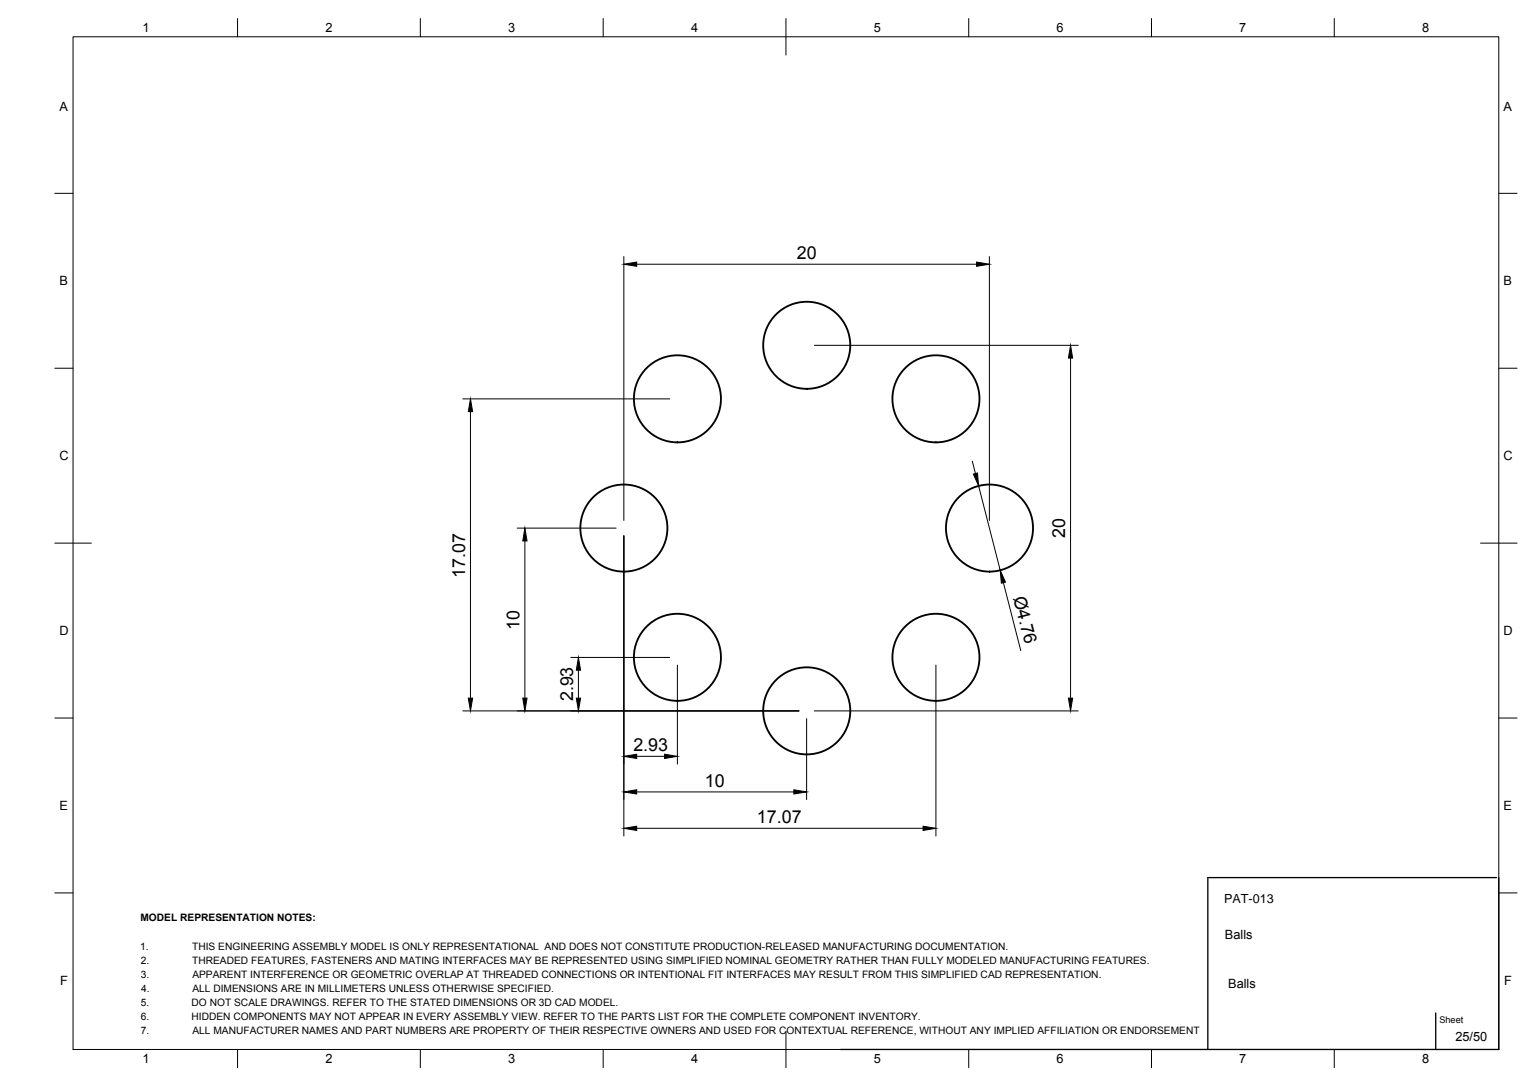
ISO-10303-21;
HEADER;
/* Generated by software containing ST-Developer
 * from STEP Tools, Inc. (www.steptools.com) 
 */

FILE_DESCRIPTION(
/* description */ ('Belt-driven linear axis on 2020 extrusion'),
/* implementation_level */ '2;1');

FILE_NAME(
/* name */ 'Balls.step',
/* time_stamp */ '2026-10-28T03:26:09-07:00',
/* author */ (''),
/* organization */ (''),
/* preprocessor_version */ 'ST-DEVELOPER v20.2',
/* originating_system */ 'Autodesk Translation Framework v15.17.0.0',
/* authorisation */ '');

FILE_SCHEMA (('AUTOMOTIVE_DESIGN { 1 0 10303 214 3 1 1 }'));
ENDSEC;

DATA;
#10=MECHANICAL_DESIGN_GEOMETRIC_PRESENTATION_REPRESENTATION('',(#628,#629,#630,#631,#632,#633,#634,#635),#20096);
#481=SPHERICAL_SURFACE('',#11958,0.23815);
#482=SPHERICAL_SURFACE('',#11960,0.23815);
#483=SPHERICAL_SURFACE('',#11962,0.23815);
#484=SPHERICAL_SURFACE('',#11964,0.23815);
#485=SPHERICAL_SURFACE('',#11966,0.23815);
#486=SPHERICAL_SURFACE('',#11968,0.23815);
#487=SPHERICAL_SURFACE('',#11970,0.23815);
#488=SPHERICAL_SURFACE('',#11972,0.23815);
#534=SHAPE_REPRESENTATION_RELATIONSHIP('SRR','None',#20331,#580);
#580=ADVANCED_BREP_SHAPE_REPRESENTATION('',(#684,#685,#686,#687,#688,#689,
#690,#691),#20062);
#628=STYLED_ITEM('',(#20650),#684);
#629=STYLED_ITEM('',(#20650),#685);
#630=STYLED_ITEM('',(#20650),#686);
#631=STYLED_ITEM('',(#20650),#687);
#632=STYLED_ITEM('',(#20650),#688);
#633=STYLED_ITEM('',(#20650),#689);
#634=STYLED_ITEM('',(#20650),#690);
#635=STYLED_ITEM('',(#20650),#691);
#684=MANIFOLD_SOLID_BREP('Body1',#10941);
#685=MANIFOLD_SOLID_BREP('Body2',#10942);
#686=MANIFOLD_SOLID_BREP('Body3',#10943);
#687=MANIFOLD_SOLID_BREP('Body4',#10944);
#688=MANIFOLD_SOLID_BREP('Body5',#10945);
#689=MANIFOLD_SOLID_BREP('Body6',#10946);
#690=MANIFOLD_SOLID_BREP('Body7',#10947);
#691=MANIFOLD_SOLID_BREP('Body8',#10948);
#1480=FACE_OUTER_BOUND('',#2192,.T.);
#1481=FACE_OUTER_BOUND('',#2193,.T.);
#1482=FACE_OUTER_BOUND('',#2194,.T.);
#1483=FACE_OUTER_BOUND('',#2195,.T.);
#1484=FACE_OUTER_BOUND('',#2196,.T.);
#1485=FACE_OUTER_BOUND('',#2197,.T.);
#1486=FACE_OUTER_BOUND('',#2198,.T.);
#1487=FACE_OUTER_BOUND('',#2199,.T.);
#2192=EDGE_LOOP('',(#8289,#8290));
#2193=EDGE_LOOP('',(#8291,#8292));
#2194=EDGE_LOOP('',(#8293,#8294));
#2195=EDGE_LOOP('',(#8295,#8296));
#2196=EDGE_LOOP('',(#8297,#8298));
#2197=EDGE_LOOP('',(#8299,#8300));
#2198=EDGE_LOOP('',(#8301,#8302));
#2199=EDGE_LOOP('',(#8303,#8304));
#4597=CIRCLE('',#11959,0.23815);
#4598=CIRCLE('',#11961,0.23815);
#4599=CIRCLE('',#11963,0.23815);
#4600=CIRCLE('',#11965,0.23815);
#4601=CIRCLE('',#11967,0.23815);
#4602=CIRCLE('',#11969,0.23815);
#4603=CIRCLE('',#11971,0.23815);
#4604=CIRCLE('',#11973,0.23815);
#5236=VERTEX_POINT('',#17345);
#5237=VERTEX_POINT('',#17346);
#5238=VERTEX_POINT('',#17349);
#5239=VERTEX_POINT('',#17350);
#5240=VERTEX_POINT('',#17353);
#5241=VERTEX_POINT('',#17354);
#5242=VERTEX_POINT('',#17357);
#5243=VERTEX_POINT('',#17358);
#5244=VERTEX_POINT('',#17361);
#5245=VERTEX_POINT('',#17362);
#5246=VERTEX_POINT('',#17365);
#5247=VERTEX_POINT('',#17366);
#5248=VERTEX_POINT('',#17369);
#5249=VERTEX_POINT('',#17370);
#5250=VERTEX_POINT('',#17373);
#5251=VERTEX_POINT('',#17374);
#6359=EDGE_CURVE('',#5236,#5237,#4597,.T.);
#6360=EDGE_CURVE('',#5238,#5239,#4598,.T.);
#6361=EDGE_CURVE('',#5240,#5241,#4599,.T.);
#6362=EDGE_CURVE('',#5242,#5243,#4600,.T.);
#6363=EDGE_CURVE('',#5244,#5245,#4601,.T.);
#6364=EDGE_CURVE('',#5246,#5247,#4602,.T.);
#6365=EDGE_CURVE('',#5248,#5249,#4603,.T.);
#6366=EDGE_CURVE('',#5250,#5251,#4604,.T.);
#8289=ORIENTED_EDGE('',*,*,#6359,.T.);
#8290=ORIENTED_EDGE('',*,*,#6359,.F.);
#8291=ORIENTED_EDGE('',*,*,#6360,.T.);
#8292=ORIENTED_EDGE('',*,*,#6360,.F.);
#8293=ORIENTED_EDGE('',*,*,#6361,.T.);
#8294=ORIENTED_EDGE('',*,*,#6361,.F.);
#8295=ORIENTED_EDGE('',*,*,#6362,.T.);
#8296=ORIENTED_EDGE('',*,*,#6362,.F.);
#8297=ORIENTED_EDGE('',*,*,#6363,.T.);
#8298=ORIENTED_EDGE('',*,*,#6363,.F.);
#8299=ORIENTED_EDGE('',*,*,#6364,.T.);
#8300=ORIENTED_EDGE('',*,*,#6364,.F.);
#8301=ORIENTED_EDGE('',*,*,#6365,.T.);
#8302=ORIENTED_EDGE('',*,*,#6365,.F.);
#8303=ORIENTED_EDGE('',*,*,#6366,.T.);
#8304=ORIENTED_EDGE('',*,*,#6366,.F.);
#10531=ADVANCED_FACE('',(#1480),#481,.T.);
#10532=ADVANCED_FACE('',(#1481),#482,.T.);
#10533=ADVANCED_FACE('',(#1482),#483,.T.);
#10534=ADVANCED_FACE('',(#1483),#484,.T.);
#10535=ADVANCED_FACE('',(#1484),#485,.T.);
#10536=ADVANCED_FACE('',(#1485),#486,.T.);
#10537=ADVANCED_FACE('',(#1486),#487,.T.);
#10538=ADVANCED_FACE('',(#1487),#488,.T.);
#10941=CLOSED_SHELL('',(#10531));
#10942=CLOSED_SHELL('',(#10532));
#10943=CLOSED_SHELL('',(#10533));
#10944=CLOSED_SHELL('',(#10534));
#10945=CLOSED_SHELL('',(#10535));
#10946=CLOSED_SHELL('',(#10536));
#10947=CLOSED_SHELL('',(#10537));
#10948=CLOSED_SHELL('',(#10538));
#11957=AXIS2_PLACEMENT_3D('',#17343,#14019,#14020);
#11958=AXIS2_PLACEMENT_3D('',#17344,#14021,#14022);
#11959=AXIS2_PLACEMENT_3D('',#17347,#14023,#14024);
#11960=AXIS2_PLACEMENT_3D('',#17348,#14025,#14026);
#11961=AXIS2_PLACEMENT_3D('',#17351,#14027,#14028);
#11962=AXIS2_PLACEMENT_3D('',#17352,#14029,#14030);
#11963=AXIS2_PLACEMENT_3D('',#17355,#14031,#14032);
#11964=AXIS2_PLACEMENT_3D('',#17356,#14033,#14034);
#11965=AXIS2_PLACEMENT_3D('',#17359,#14035,#14036);
#11966=AXIS2_PLACEMENT_3D('',#17360,#14037,#14038);
#11967=AXIS2_PLACEMENT_3D('',#17363,#14039,#14040);
#11968=AXIS2_PLACEMENT_3D('',#17364,#14041,#14042);
#11969=AXIS2_PLACEMENT_3D('',#17367,#14043,#14044);
#11970=AXIS2_PLACEMENT_3D('',#17368,#14045,#14046);
#11971=AXIS2_PLACEMENT_3D('',#17371,#14047,#14048);
#11972=AXIS2_PLACEMENT_3D('',#17372,#14049,#14050);
#11973=AXIS2_PLACEMENT_3D('',#17375,#14051,#14052);
#14019=DIRECTION('axis',(0.,0.,1.));
#14020=DIRECTION('refdir',(1.,0.,0.));
#14021=DIRECTION('center_axis',(0.,0.,1.));
#14022=DIRECTION('ref_axis',(1.,0.,0.));
#14023=DIRECTION('center_axis',(1.22464679914735E-16,-1.,0.));
#14024=DIRECTION('ref_axis',(-1.,-1.22464679914735E-16,0.));
#14025=DIRECTION('center_axis',(0.707106781186548,0.,0.707106781186548));
#14026=DIRECTION('ref_axis',(0.707106781186548,0.,-0.707106781186548));
#14027=DIRECTION('center_axis',(8.65956056235494E-17,-1.,-8.65956056235493E-17));
#14028=DIRECTION('ref_axis',(-0.707106781186547,-1.22464679914735E-16,0.707106781186547));
#14029=DIRECTION('center_axis',(1.,0.,0.));
#14030=DIRECTION('ref_axis',(6.12323399573676E-17,0.,-1.));
#14031=DIRECTION('center_axis',(7.49879891330929E-33,-1.,-1.22464679914735E-16));
#14032=DIRECTION('ref_axis',(-6.12323399573676E-17,-1.22464679914735E-16,
1.));
#14033=DIRECTION('center_axis',(0.707106781186548,0.,-0.707106781186548));
#14034=DIRECTION('ref_axis',(-0.707106781186548,0.,-0.707106781186548));
#14035=DIRECTION('center_axis',(-8.65956056235493E-17,-1.,-8.65956056235494E-17));
#14036=DIRECTION('ref_axis',(0.707106781186547,-1.22464679914735E-16,0.707106781186547));
#14037=DIRECTION('center_axis',(0.,0.,-1.));
#14038=DIRECTION('ref_axis',(-1.,0.,-1.22464679914735E-16));
#14039=DIRECTION('center_axis',(-1.22464679914735E-16,-1.,-1.49975978266186E-32));
#14040=DIRECTION('ref_axis',(1.,-1.22464679914735E-16,1.22464679914735E-16));
#14041=DIRECTION('center_axis',(-0.707106781186547,0.,-0.707106781186548));
#14042=DIRECTION('ref_axis',(-0.707106781186548,0.,0.707106781186547));
#14043=DIRECTION('center_axis',(-8.65956056235493E-17,-1.,8.65956056235493E-17));
#14044=DIRECTION('ref_axis',(0.707106781186548,-1.22464679914735E-16,-0.707106781186547));
#14045=DIRECTION('center_axis',(-1.,0.,0.));
#14046=DIRECTION('ref_axis',(-1.83697019872103E-16,0.,1.));
#14047=DIRECTION('center_axis',(-2.24963967399279E-32,-1.,1.22464679914735E-16));
#14048=DIRECTION('ref_axis',(1.83697019872103E-16,-1.22464679914735E-16,
-1.));
#14049=DIRECTION('center_axis',(-0.707106781186548,0.,0.707106781186548));
#14050=DIRECTION('ref_axis',(0.707106781186547,0.,0.707106781186548));
#14051=DIRECTION('center_axis',(8.65956056235493E-17,-1.,8.65956056235493E-17));
#14052=DIRECTION('ref_axis',(-0.707106781186547,-1.22464679914735E-16,-0.707106781186548));
#17343=CARTESIAN_POINT('',(0.,0.,0.));
#17344=CARTESIAN_POINT('Origin',(1.,0.,0.));
#17345=CARTESIAN_POINT('',(1.,-1.78583896120461E-33,0.23815));
#17346=CARTESIAN_POINT('',(1.,-1.78583896120461E-33,-0.23815));
#17347=CARTESIAN_POINT('Origin',(1.,0.,0.));
#17348=CARTESIAN_POINT('Origin',(0.707106781186548,0.,-0.707106781186547));
#17349=CARTESIAN_POINT('',(0.875504261126124,-1.78583896120461E-33,-0.538709301246971));
#17350=CARTESIAN_POINT('',(0.538709301246971,-1.78583896120461E-33,-0.875504261126124));
#17351=CARTESIAN_POINT('Origin',(0.707106781186548,0.,-0.707106781186547));
#17352=CARTESIAN_POINT('Origin',(6.12323399573677E-17,0.,-1.));
#17353=CARTESIAN_POINT('',(0.23815,-1.78583896120461E-33,-1.));
#17354=CARTESIAN_POINT('',(-0.23815,-1.78583896120461E-33,-1.));
#17355=CARTESIAN_POINT('Origin',(6.12323399573677E-17,0.,-1.));
#17356=CARTESIAN_POINT('Origin',(-0.707106781186547,0.,-0.707106781186548));
#17357=CARTESIAN_POINT('',(-0.538709301246971,-1.78583896120461E-33,-0.875504261126124));
#17358=CARTESIAN_POINT('',(-0.875504261126124,-1.78583896120461E-33,-0.538709301246971));
#17359=CARTESIAN_POINT('Origin',(-0.707106781186547,0.,-0.707106781186548));
#17360=CARTESIAN_POINT('Origin',(-1.,0.,-1.22464679914735E-16));
#17361=CARTESIAN_POINT('',(-1.,-1.78583896120461E-33,-0.23815));
#17362=CARTESIAN_POINT('',(-1.,-1.78583896120461E-33,0.23815));
#17363=CARTESIAN_POINT('Origin',(-1.,0.,-1.22464679914735E-16));
#17364=CARTESIAN_POINT('Origin',(-0.707106781186548,0.,0.707106781186547));
#17365=CARTESIAN_POINT('',(-0.875504261126124,-7.94881478324376E-33,0.538709301246971));
#17366=CARTESIAN_POINT('',(-0.538709301246971,4.37713686083455E-33,0.875504261126124));
#17367=CARTESIAN_POINT('Origin',(-0.707106781186548,0.,0.707106781186547));
#17368=CARTESIAN_POINT('Origin',(-1.83697019872103E-16,0.,1.));
#17369=CARTESIAN_POINT('',(-0.23815,-1.78583896120461E-33,1.));
#17370=CARTESIAN_POINT('',(0.23815,-1.78583896120461E-33,1.));
#17371=CARTESIAN_POINT('Origin',(-1.83697019872103E-16,0.,1.));
#17372=CARTESIAN_POINT('Origin',(0.707106781186547,0.,0.707106781186548));
#17373=CARTESIAN_POINT('',(0.538709301246971,-4.86732687222419E-33,0.875504261126124));
#17374=CARTESIAN_POINT('',(0.875504261126124,1.29564894981497E-33,0.538709301246971));
#17375=CARTESIAN_POINT('Origin',(0.707106781186547,0.,0.707106781186548));
#20008=UNCERTAINTY_MEASURE_WITH_UNIT(LENGTH_MEASURE(0.001),#20097,
'DISTANCE_ACCURACY_VALUE',
'Maximum model space distance between geometric entities at asserted c
onnectivities');
#20042=UNCERTAINTY_MEASURE_WITH_UNIT(LENGTH_MEASURE(0.001),#20097,
'DISTANCE_ACCURACY_VALUE',
'Maximum model space distance between geometric entities at asserted c
onnectivities');
#20062=(
GEOMETRIC_REPRESENTATION_CONTEXT(3)
GLOBAL_UNCERTAINTY_ASSIGNED_CONTEXT((#20008))
GLOBAL_UNIT_ASSIGNED_CONTEXT((#20097,#20099,#20100))
REPRESENTATION_CONTEXT('','3D')
);
#20096=(
GEOMETRIC_REPRESENTATION_CONTEXT(3)
GLOBAL_UNCERTAINTY_ASSIGNED_CONTEXT((#20042))
GLOBAL_UNIT_ASSIGNED_CONTEXT((#20097,#20099,#20100))
REPRESENTATION_CONTEXT('','3D')
);
#20097=(
LENGTH_UNIT()
NAMED_UNIT(*)
SI_UNIT(.CENTI.,.METRE.)
);
#20099=(
NAMED_UNIT(*)
PLANE_ANGLE_UNIT()
SI_UNIT($,.RADIAN.)
);
#20100=(
NAMED_UNIT(*)
SI_UNIT($,.STERADIAN.)
SOLID_ANGLE_UNIT()
);
#20120=SHAPE_DEFINITION_REPRESENTATION(#20173,#20331);
#20173=PRODUCT_DEFINITION_SHAPE('',$,#20385);
#20331=SHAPE_REPRESENTATION('',(#11957),#20062);
#20365=PRODUCT_DEFINITION_CONTEXT('part definition',#20526,'design');
#20385=PRODUCT_DEFINITION('Balls','Balls',#20438,#20365);
#20438=PRODUCT_DEFINITION_FORMATION('',$,#20547);
#20526=APPLICATION_CONTEXT(
'Core Data for Automotive Mechanical Design Process');
#20527=PRODUCT_CONTEXT('part definition',#20526,'mechanical');
#20547=PRODUCT('Balls','Balls','Balls',(#20527));
#20644=COLOUR_RGB('Grey',0.48,0.52,0.57);
#20645=FILL_AREA_STYLE_COLOUR('',#20644);
#20646=FILL_AREA_STYLE('',(#20645));
#20647=SURFACE_STYLE_FILL_AREA(#20646);
#20648=SURFACE_SIDE_STYLE('',(#20647));
#20649=SURFACE_STYLE_USAGE(.BOTH.,#20648);
#20650=PRESENTATION_STYLE_ASSIGNMENT((#20649));
ENDSEC;
END-ISO-10303-21;
